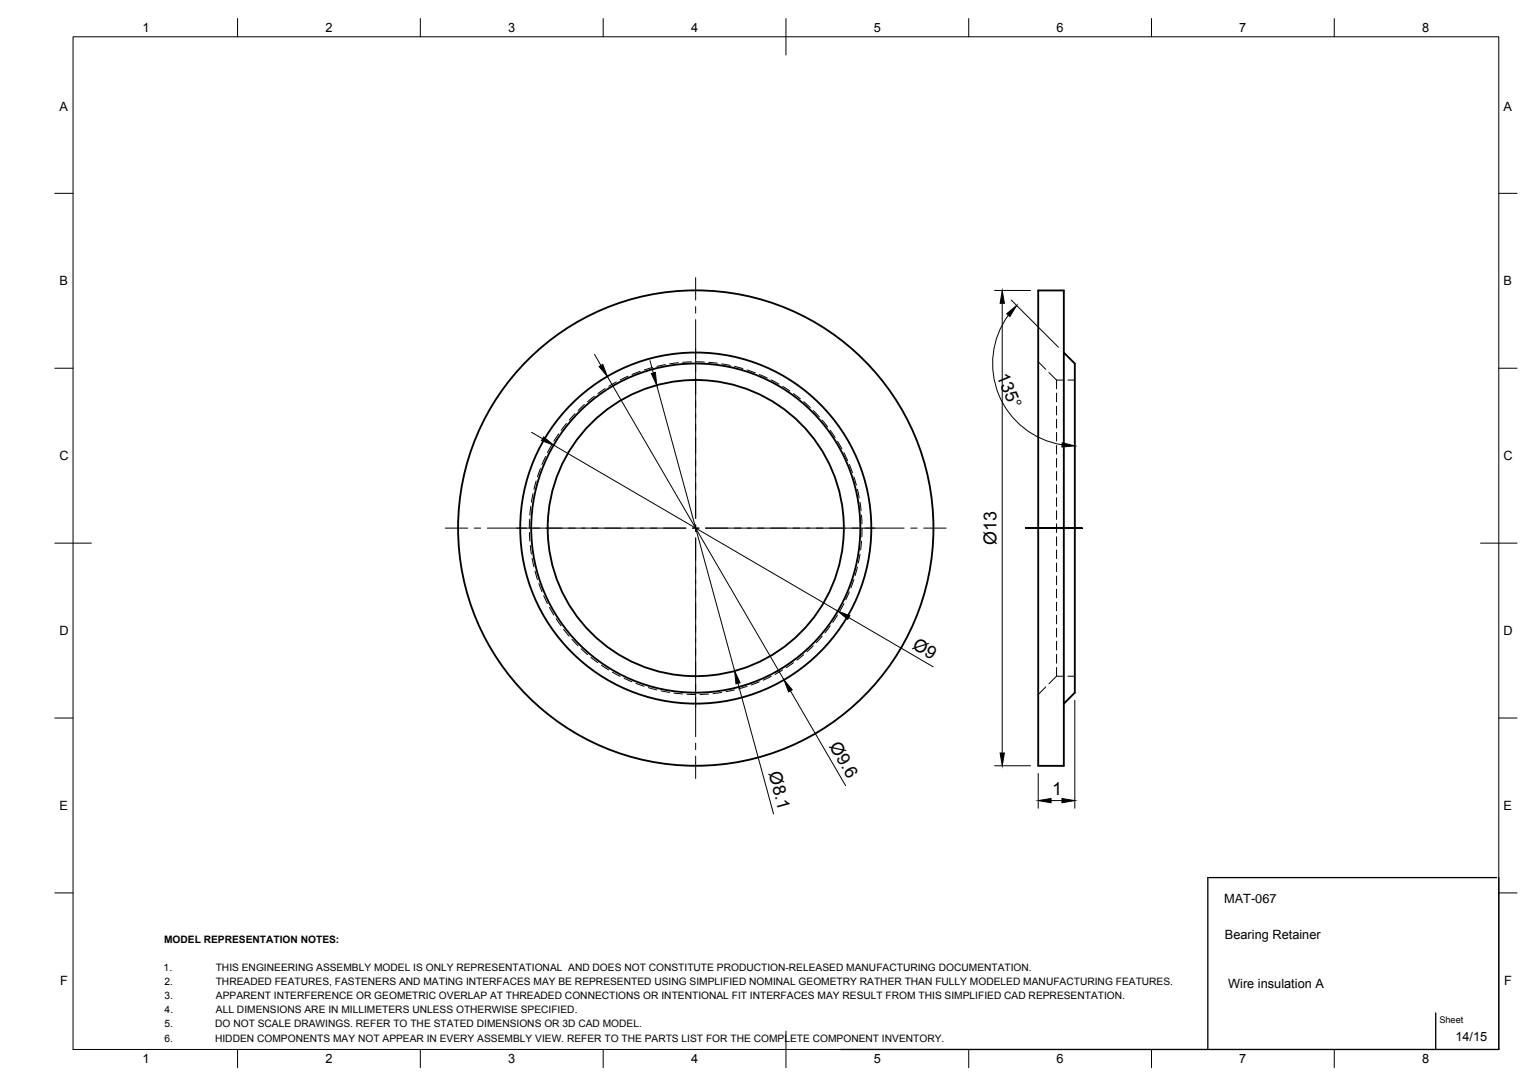
ISO-10303-21;
HEADER;
/* Generated by software containing ST-Developer
 * from STEP Tools, Inc. (www.steptools.com) 
 */

FILE_DESCRIPTION(
/* description */ ('CAx-IF Rec.Pracs.---Representation and Presentation of Product Manufa
cturing Information (PMI)---4.0---2014-10-13'),
/* implementation_level */ '2;1');

FILE_NAME(
/* name */ 'Bearing Retainer.step',
/* time_stamp */ '2026-10-24T16:02:03-07:00',
/* author */ (''),
/* organization */ (''),
/* preprocessor_version */ 'ST-DEVELOPER v20.2',
/* originating_system */ 'Autodesk Translation Framework v15.17.0.0',
/* authorisation */ '');

FILE_SCHEMA (('AP242_MANAGED_MODEL_BASED_3D_ENGINEERING_MIM_LF { 1 0 10303 442 2 1 4 }'));
ENDSEC;

DATA;
#10=MECHANICAL_DESIGN_GEOMETRIC_PRESENTATION_REPRESENTATION('',(#358),#6348);
#323=CONICAL_SURFACE('',#3888,0.0043,0.785398163397448);
#324=CONICAL_SURFACE('',#3894,0.0046499998960644,0.785398163397448);
#336=SHAPE_REPRESENTATION_RELATIONSHIP('SRR','None',#6498,#347);
#347=ADVANCED_BREP_SHAPE_REPRESENTATION('',(#369),#6346);
#358=STYLED_ITEM('',(#6604),#369);
#369=MANIFOLD_SOLID_BREP('Body1',#3397);
#460=CYLINDRICAL_SURFACE('',#3884,0.0065);
#461=CYLINDRICAL_SURFACE('',#3890,0.00405);
#501=FACE_BOUND('',#1063,.T.);
#502=FACE_BOUND('',#1066,.T.);
#503=FACE_BOUND('',#1070,.T.);
#683=CIRCLE('',#3882,0.00650000000001);
#684=CIRCLE('',#3883,0.00479999989272164);
#685=CIRCLE('',#3885,0.00650000000001);
#686=CIRCLE('',#3887,0.00455000000001);
#687=CIRCLE('',#3889,0.00405000000001);
#688=CIRCLE('',#3891,0.00405000000001);
#689=CIRCLE('',#3893,0.00449999989942716);
#854=FACE_OUTER_BOUND('',#1062,.T.);
#855=FACE_OUTER_BOUND('',#1064,.T.);
#856=FACE_OUTER_BOUND('',#1065,.T.);
#857=FACE_OUTER_BOUND('',#1067,.T.);
#858=FACE_OUTER_BOUND('',#1068,.T.);
#859=FACE_OUTER_BOUND('',#1069,.T.);
#860=FACE_OUTER_BOUND('',#1071,.T.);
#1062=EDGE_LOOP('',(#3103));
#1063=EDGE_LOOP('',(#3104));
#1064=EDGE_LOOP('',(#3105,#3106,#3107,#3108));
#1065=EDGE_LOOP('',(#3109));
#1066=EDGE_LOOP('',(#3110));
#1067=EDGE_LOOP('',(#3111,#3112,#3113,#3114));
#1068=EDGE_LOOP('',(#3115,#3116,#3117,#3118));
#1069=EDGE_LOOP('',(#3119));
#1070=EDGE_LOOP('',(#3120));
#1071=EDGE_LOOP('',(#3121,#3122,#3123,#3124));
#1305=LINE('',#6191,#1538);
#1306=LINE('',#6198,#1539);
#1307=LINE('',#6202,#1540);
#1308=LINE('',#6207,#1541);
#1538=VECTOR('',#4937,0.0065);
#1539=VECTOR('',#4946,0.0043);
#1540=VECTOR('',#4951,0.00405);
#1541=VECTOR('',#4958,0.0046499998960644);
#1821=VERTEX_POINT('',#6184);
#1822=VERTEX_POINT('',#6186);
#1823=VERTEX_POINT('',#6189);
#1824=VERTEX_POINT('',#6193);
#1825=VERTEX_POINT('',#6196);
#1826=VERTEX_POINT('',#6200);
#1827=VERTEX_POINT('',#6204);
#2250=EDGE_CURVE('',#1821,#1821,#683,.T.);
#2251=EDGE_CURVE('',#1822,#1822,#684,.T.);
#2252=EDGE_CURVE('',#1823,#1823,#685,.T.);
#2253=EDGE_CURVE('',#1823,#1821,#1305,.T.);
#2254=EDGE_CURVE('',#1824,#1824,#686,.T.);
#2255=EDGE_CURVE('',#1825,#1825,#687,.T.);
#2256=EDGE_CURVE('',#1825,#1824,#1306,.T.);
#2257=EDGE_CURVE('',#1826,#1826,#688,.T.);
#2258=EDGE_CURVE('',#1826,#1825,#1307,.T.);
#2259=EDGE_CURVE('',#1827,#1827,#689,.T.);
#2260=EDGE_CURVE('',#1822,#1827,#1308,.T.);
#3103=ORIENTED_EDGE('',*,*,#2250,.F.);
#3104=ORIENTED_EDGE('',*,*,#2251,.T.);
#3105=ORIENTED_EDGE('',*,*,#2252,.F.);
#3106=ORIENTED_EDGE('',*,*,#2253,.T.);
#3107=ORIENTED_EDGE('',*,*,#2250,.T.);
#3108=ORIENTED_EDGE('',*,*,#2253,.F.);
#3109=ORIENTED_EDGE('',*,*,#2252,.T.);
#3110=ORIENTED_EDGE('',*,*,#2254,.F.);
#3111=ORIENTED_EDGE('',*,*,#2255,.F.);
#3112=ORIENTED_EDGE('',*,*,#2256,.T.);
#3113=ORIENTED_EDGE('',*,*,#2254,.T.);
#3114=ORIENTED_EDGE('',*,*,#2256,.F.);
#3115=ORIENTED_EDGE('',*,*,#2257,.F.);
#3116=ORIENTED_EDGE('',*,*,#2258,.T.);
#3117=ORIENTED_EDGE('',*,*,#2255,.T.);
#3118=ORIENTED_EDGE('',*,*,#2258,.F.);
#3119=ORIENTED_EDGE('',*,*,#2259,.F.);
#3120=ORIENTED_EDGE('',*,*,#2257,.T.);
#3121=ORIENTED_EDGE('',*,*,#2251,.F.);
#3122=ORIENTED_EDGE('',*,*,#2260,.T.);
#3123=ORIENTED_EDGE('',*,*,#2259,.T.);
#3124=ORIENTED_EDGE('',*,*,#2260,.F.);
#3212=PLANE('',#3881);
#3213=PLANE('',#3886);
#3214=PLANE('',#3892);
#3377=ADVANCED_FACE('',(#854,#501),#3212,.T.);
#3378=ADVANCED_FACE('',(#855),#460,.T.);
#3379=ADVANCED_FACE('',(#856,#502),#3213,.T.);
#3380=ADVANCED_FACE('',(#857),#323,.F.);
#3381=ADVANCED_FACE('',(#858),#461,.F.);
#3382=ADVANCED_FACE('',(#859,#503),#3214,.T.);
#3383=ADVANCED_FACE('',(#860),#324,.T.);
#3397=CLOSED_SHELL('',(#3377,#3378,#3379,#3380,#3381,#3382,#3383));
#3880=AXIS2_PLACEMENT_3D('',#6182,#4925,#4926);
#3881=AXIS2_PLACEMENT_3D('',#6183,#4927,#4928);
#3882=AXIS2_PLACEMENT_3D('',#6185,#4929,#4930);
#3883=AXIS2_PLACEMENT_3D('',#6187,#4931,#4932);
#3884=AXIS2_PLACEMENT_3D('',#6188,#4933,#4934);
#3885=AXIS2_PLACEMENT_3D('',#6190,#4935,#4936);
#3886=AXIS2_PLACEMENT_3D('',#6192,#4938,#4939);
#3887=AXIS2_PLACEMENT_3D('',#6194,#4940,#4941);
#3888=AXIS2_PLACEMENT_3D('',#6195,#4942,#4943);
#3889=AXIS2_PLACEMENT_3D('',#6197,#4944,#4945);
#3890=AXIS2_PLACEMENT_3D('',#6199,#4947,#4948);
#3891=AXIS2_PLACEMENT_3D('',#6201,#4949,#4950);
#3892=AXIS2_PLACEMENT_3D('',#6203,#4952,#4953);
#3893=AXIS2_PLACEMENT_3D('',#6205,#4954,#4955);
#3894=AXIS2_PLACEMENT_3D('',#6206,#4956,#4957);
#4925=DIRECTION('axis',(0.,0.,1.));
#4926=DIRECTION('refdir',(1.,0.,0.));
#4927=DIRECTION('center_axis',(0.,-1.,0.));
#4928=DIRECTION('ref_axis',(0.,0.,-1.));
#4929=DIRECTION('center_axis',(0.,1.,0.));
#4930=DIRECTION('ref_axis',(1.,0.,0.));
#4931=DIRECTION('center_axis',(0.,1.,0.));
#4932=DIRECTION('ref_axis',(1.,0.,0.));
#4933=DIRECTION('center_axis',(0.,1.,0.));
#4934=DIRECTION('ref_axis',(0.,0.,1.));
#4935=DIRECTION('center_axis',(0.,1.,0.));
#4936=DIRECTION('ref_axis',(1.,0.,0.));
#4937=DIRECTION('',(0.,-1.,0.));
#4938=DIRECTION('center_axis',(0.,1.,0.));
#4939=DIRECTION('ref_axis',(1.,0.,0.));
#4940=DIRECTION('center_axis',(0.,1.,0.));
#4941=DIRECTION('ref_axis',(1.,0.,0.));
#4942=DIRECTION('center_axis',(0.,1.,0.));
#4943=DIRECTION('ref_axis',(0.,0.,1.));
#4944=DIRECTION('center_axis',(0.,1.,0.));
#4945=DIRECTION('ref_axis',(1.,0.,0.));
#4946=DIRECTION('',(-8.65956056235493E-17,0.707106781186548,-0.707106781186547));
#4947=DIRECTION('center_axis',(0.,1.,0.));
#4948=DIRECTION('ref_axis',(0.,0.,1.));
#4949=DIRECTION('center_axis',(0.,1.,0.));
#4950=DIRECTION('ref_axis',(1.,0.,0.));
#4951=DIRECTION('',(0.,1.,0.));
#4952=DIRECTION('center_axis',(0.,-1.,0.));
#4953=DIRECTION('ref_axis',(0.,0.,-1.));
#4954=DIRECTION('center_axis',(0.,1.,0.));
#4955=DIRECTION('ref_axis',(1.,0.,0.));
#4956=DIRECTION('center_axis',(0.,1.,0.));
#4957=DIRECTION('ref_axis',(0.,0.,1.));
#4958=DIRECTION('',(8.65956056235493E-17,-0.707106781186548,0.707106781186547));
#6182=CARTESIAN_POINT('',(0.,0.,0.));
#6183=CARTESIAN_POINT('Origin',(0.,-0.0116999997384846,0.0065));
#6184=CARTESIAN_POINT('',(-7.9602041944578E-19,-0.0116999997384946,-0.0065));
#6185=CARTESIAN_POINT('Origin',(0.,-0.0116999997384946,0.));
#6186=CARTESIAN_POINT('',(-5.87830450451699E-19,-0.0116999997384846,-0.00479999989271167));
#6187=CARTESIAN_POINT('Origin',(0.,-0.0116999997384946,0.));
#6188=CARTESIAN_POINT('Origin',(0.,-0.0113499997351319,0.));
#6189=CARTESIAN_POINT('',(-7.9602041944578E-19,-0.0109999997317891,-0.0065));
#6190=CARTESIAN_POINT('Origin',(0.,-0.0109999997317891,0.));
#6191=CARTESIAN_POINT('',(-7.9602041944578E-19,-0.0113499997351319,-0.0065));
#6192=CARTESIAN_POINT('Origin',(0.,-0.0109999997317791,0.00455));
#6193=CARTESIAN_POINT('',(-5.57214293612046E-19,-0.0109999997317791,-0.00455));
#6194=CARTESIAN_POINT('Origin',(0.,-0.0109999997317891,0.));
#6195=CARTESIAN_POINT('Origin',(0.,-0.0112499997317791,0.));
#6196=CARTESIAN_POINT('',(-4.95981953654678E-19,-0.0114999997317791,-0.00405));
#6197=CARTESIAN_POINT('Origin',(0.,-0.0114999997317891,0.));
#6198=CARTESIAN_POINT('',(-5.26598123633362E-19,-0.0112499997317791,-0.0043));
#6199=CARTESIAN_POINT('Origin',(0.,-0.0117499997317791,0.));
#6200=CARTESIAN_POINT('',(-4.95981953654678E-19,-0.0119999997317891,-0.00405));
#6201=CARTESIAN_POINT('Origin',(0.,-0.0119999997317891,0.));
#6202=CARTESIAN_POINT('',(-4.95981953654678E-19,-0.0117499997317791,-0.00405));
#6203=CARTESIAN_POINT('Origin',(0.,-0.0119999997317791,0.00449999989941716));
#6204=CARTESIAN_POINT('',(-5.51091047298466E-19,-0.0119999997317791,-0.00449999989941718));
#6205=CARTESIAN_POINT('Origin',(0.,-0.0119999997317891,0.));
#6206=CARTESIAN_POINT('Origin',(0.,-0.0118499997351319,0.));
#6207=CARTESIAN_POINT('',(-5.69460748875079E-19,-0.0118499997351319,-0.0046499998960644));
#6321=UNCERTAINTY_MEASURE_WITH_UNIT(LENGTH_MEASURE(1.E-5),#6349,
'DISTANCE_ACCURACY_VALUE',
'Maximum model space distance between geometric entities at asserted c
onnectivities');
#6323=UNCERTAINTY_MEASURE_WITH_UNIT(LENGTH_MEASURE(1.E-5),#6349,
'DISTANCE_ACCURACY_VALUE',
'Maximum model space distance between geometric entities at asserted c
onnectivities');
#6346=(
GEOMETRIC_REPRESENTATION_CONTEXT(3)
GLOBAL_UNCERTAINTY_ASSIGNED_CONTEXT((#6321))
GLOBAL_UNIT_ASSIGNED_CONTEXT((#6349,#6350,#6351))
REPRESENTATION_CONTEXT('','3D')
);
#6348=(
GEOMETRIC_REPRESENTATION_CONTEXT(3)
GLOBAL_UNCERTAINTY_ASSIGNED_CONTEXT((#6323))
GLOBAL_UNIT_ASSIGNED_CONTEXT((#6349,#6350,#6351))
REPRESENTATION_CONTEXT('','3D')
);
#6349=(
LENGTH_UNIT()
NAMED_UNIT(*)
SI_UNIT($,.METRE.)
);
#6350=(
NAMED_UNIT(*)
PLANE_ANGLE_UNIT()
SI_UNIT($,.RADIAN.)
);
#6351=(
NAMED_UNIT(*)
SI_UNIT($,.STERADIAN.)
SOLID_ANGLE_UNIT()
);
#6374=SHAPE_DEFINITION_REPRESENTATION(#6398,#6498);
#6398=PRODUCT_DEFINITION_SHAPE('',$,#6523);
#6498=SHAPE_REPRESENTATION('',(#3880),#6346);
#6500=PRODUCT_DEFINITION_CONTEXT('part definition',#6574,'design');
#6523=PRODUCT_DEFINITION('Bearing Retainer','Bearing Retainer',#6547,#6500);
#6547=PRODUCT_DEFINITION_FORMATION('',$,#6598);
#6574=APPLICATION_CONTEXT('Managed model based 3d engineering');
#6575=PRODUCT_CONTEXT('part definition',#6574,'mechanical');
#6598=PRODUCT('Bearing Retainer','Bearing Retainer',
'LEGAL AND USAGE DISCLAIMER: this Data/Model is provided \X2\201C\X0\A
S IS\X2\201D\X0\ for informational and representational only. It is a 
geometric approximation and is NOT engineered, certified, or guarantee
d for dimensional accuracy, exact tolerances, or production-level prec
ision. Vendor disclaims all implied warranties including fitness for a
 particular purpose. DO NOT USE FOR DIRECT PHYSICAL MANUFACTURING, AUT
OMATED PRODUCTION, OR SAFETY-CRITICAL SYSTEMS without independent engi
neering verification and resolution of any design discrepancies.',(#6575));
#6604=PRESENTATION_STYLE_ASSIGNMENT((#6610));
#6610=SURFACE_STYLE_USAGE(.BOTH.,#6616);
#6616=SURFACE_SIDE_STYLE('',(#6622));
#6622=SURFACE_STYLE_FILL_AREA(#6628);
#6628=FILL_AREA_STYLE('Opaque(25,25,25)',(#6634));
#6634=FILL_AREA_STYLE_COLOUR('Opaque(25,25,25)',#6640);
#6640=COLOUR_RGB('Opaque(25,25,25)',0.0980392156862745,0.0980392156862745,
0.0980392156862745);
ENDSEC;
END-ISO-10303-21;
